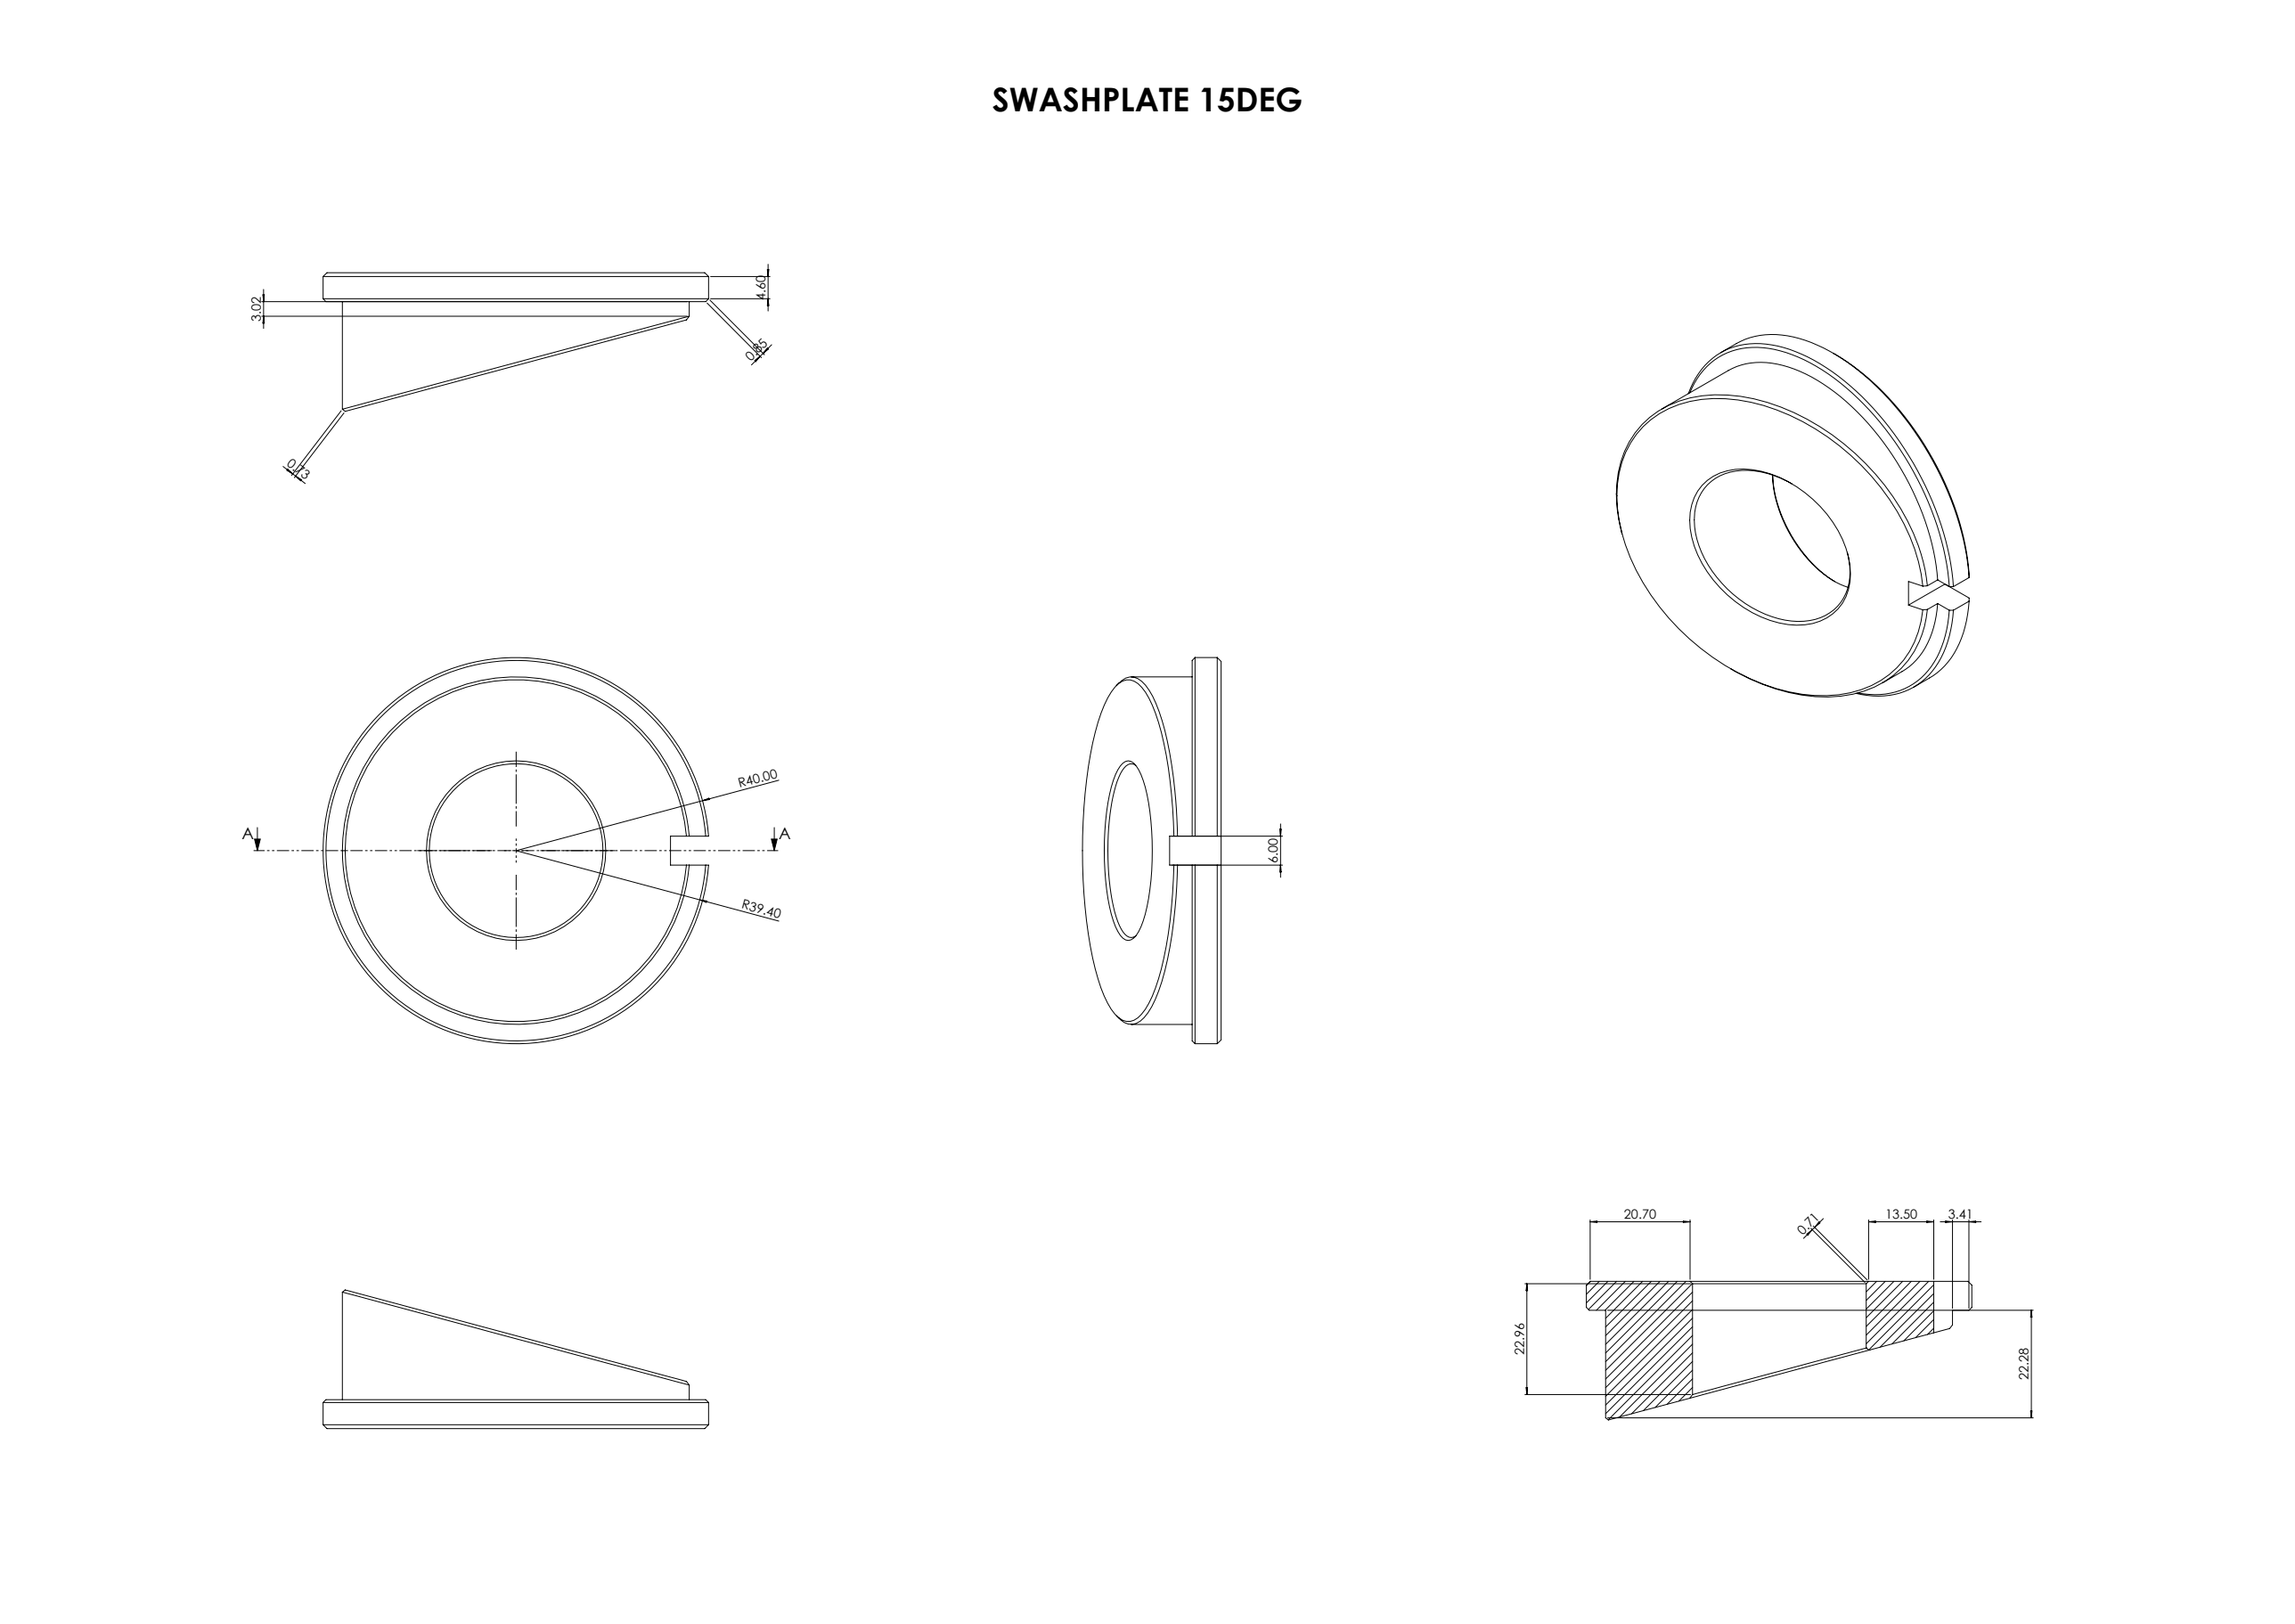
ISO-10303-21;
HEADER;
/* Generated by software containing ST-Developer
 * from STEP Tools, Inc. (www.steptools.com) 
 */

FILE_DESCRIPTION(
/* description */ (''),
/* implementation_level */ '2;1');

FILE_NAME(
/* name */ '10_Swashplate_15deg.step',
/* time_stamp */ '2026-10-23T00:52:27+05:00',
/* author */ (''),
/* organization */ (''),
/* preprocessor_version */ 'ST-DEVELOPER v20.2',
/* originating_system */ 'Autodesk Translation Framework v15.15.0.0',
/* authorisation */ '');

FILE_SCHEMA (('AUTOMOTIVE_DESIGN { 1 0 10303 214 3 1 1 }'));
ENDSEC;

DATA;
#10=MECHANICAL_DESIGN_GEOMETRIC_PRESENTATION_REPRESENTATION('',(#1550),#59204);
#314=B_SPLINE_SURFACE_WITH_KNOTS('',3,3,((#30941,#30942,#30943,#30944,#30945,
#30946,#30947,#30948,#30949,#30950),(#30951,#30952,#30953,#30954,#30955,
#30956,#30957,#30958,#30959,#30960),(#30961,#30962,#30963,#30964,#30965,
#30966,#30967,#30968,#30969,#30970),(#30971,#30972,#30973,#30974,#30975,
#30976,#30977,#30978,#30979,#30980)),.UNSPECIFIED.,.F.,.F.,.F.,(4,4),(4,
1,1,1,1,1,1,4),(0.,1.),(0.0830596749235681,0.519992957590172,0.956926240256775,
1.39385952292338,1.83079280558998,2.26772608825659,2.70465937092319,3.14159265358979),
 .UNSPECIFIED.);
#315=B_SPLINE_SURFACE_WITH_KNOTS('',3,3,((#31030,#31031,#31032,#31033,#31034,
#31035,#31036,#31037,#31038,#31039),(#31040,#31041,#31042,#31043,#31044,
#31045,#31046,#31047,#31048,#31049),(#31050,#31051,#31052,#31053,#31054,
#31055,#31056,#31057,#31058,#31059),(#31060,#31061,#31062,#31063,#31064,
#31065,#31066,#31067,#31068,#31069)),.UNSPECIFIED.,.F.,.F.,.F.,(4,4),(4,
1,1,1,1,1,1,4),(0.,1.),(-3.14159265358979,-2.70465937092292,-2.26772608825605,
-1.83079280558918,-1.39385952292231,-0.95692624025544,-0.519992957588569,
-0.083059674921698),.UNSPECIFIED.);
#316=B_SPLINE_SURFACE_WITH_KNOTS('',3,3,((#31111,#31112,#31113,#31114,#31115,
#31116,#31117,#31118,#31119,#31120,#31121,#31122,#31123,#31124,#31125,#31126,
#31127),(#31128,#31129,#31130,#31131,#31132,#31133,#31134,#31135,#31136,
#31137,#31138,#31139,#31140,#31141,#31142,#31143,#31144),(#31145,#31146,
#31147,#31148,#31149,#31150,#31151,#31152,#31153,#31154,#31155,#31156,#31157,
#31158,#31159,#31160,#31161),(#31162,#31163,#31164,#31165,#31166,#31167,
#31168,#31169,#31170,#31171,#31172,#31173,#31174,#31175,#31176,#31177,#31178)),
 .UNSPECIFIED.,.F.,.T.,.F.,(4,4),(4,1,1,1,1,1,1,1,1,1,1,1,1,1,4),(0.,1.),
(-3.14159265358979,-2.69279370307697,-2.24399475256414,-1.79519580205131,
-1.34639685153848,-1.0471975511966,-0.448798950512828,-0.149599650170943,
0.448798950512828,0.747998250854713,1.34639685153848,1.64559615188037,2.24399475256414,
2.69279370307697,3.14159265358979),.UNSPECIFIED.);
#569=B_SPLINE_CURVE_WITH_KNOTS('',3,(#30893,#30894,#30895,#30896,#30897,
#30898),.UNSPECIFIED.,.F.,.F.,(4,2,4),(-0.0953956468456381,-0.0476986988383283,
0.),.UNSPECIFIED.);
#570=B_SPLINE_CURVE_WITH_KNOTS('',3,(#30921,#30922,#30923,#30924,#30925,
#30926),.UNSPECIFIED.,.F.,.F.,(4,2,4),(-0.0953955489316151,-0.0476968906569989,
0.),.UNSPECIFIED.);
#571=B_SPLINE_CURVE_WITH_KNOTS('',3,(#30982,#30983,#30984,#30985,#30986,
#30987,#30988,#30989,#30990,#30991),.UNSPECIFIED.,.F.,.F.,(4,1,1,1,1,1,
1,4),(0.0848980286013396,0.519992957590172,0.956926240256775,1.39385952292338,
1.83079280558998,2.26772608825659,2.70465937092319,3.14159265358979),
 .UNSPECIFIED.);
#572=B_SPLINE_CURVE_WITH_KNOTS('',3,(#30994,#30995,#30996,#30997,#30998,
#30999,#31000,#31001,#31002,#31003),.UNSPECIFIED.,.F.,.F.,(4,1,1,1,1,1,
1,4),(-3.14159265358979,-2.70465937092319,-2.26772608825659,-1.83079280558998,
-1.39385952292338,-0.956926240256775,-0.519992957590172,-0.0830596749235681),
 .UNSPECIFIED.);
#573=B_SPLINE_CURVE_WITH_KNOTS('',3,(#31012,#31013,#31014,#31015,#31016,
#31017,#31018,#31019,#31020,#31021,#31022,#31023,#31024,#31025,#31026,#31027,
#31028),.UNSPECIFIED.,.T.,.F.,(4,1,1,1,1,1,1,1,1,1,1,1,1,1,4),(-3.14159265358979,
-2.69279370307697,-2.24399475256414,-1.64559615188037,-1.34639685153848,
-0.747998250854713,-0.448798950512828,0.149599650170943,0.448798950512828,
1.0471975511966,1.34639685153848,1.79519580205131,2.24399475256414,2.69279370307697,
3.14159265358979),.UNSPECIFIED.);
#574=B_SPLINE_CURVE_WITH_KNOTS('',3,(#31070,#31071,#31072,#31073,#31074,
#31075,#31076,#31077,#31078,#31079),.UNSPECIFIED.,.F.,.F.,(4,1,1,1,1,1,
1,4),(0.083059674921698,0.519992957588569,0.95692624025544,1.39385952292231,
1.83079280558918,2.26772608825605,2.70465937092292,3.14159265358979),
 .UNSPECIFIED.);
#575=B_SPLINE_CURVE_WITH_KNOTS('',3,(#31080,#31081,#31082,#31083,#31084,
#31085,#31086,#31087,#31088,#31089),.UNSPECIFIED.,.F.,.F.,(4,1,1,1,1,1,
1,4),(-3.14159265358979,-2.70465937092292,-2.26772608825605,-1.83079280558918,
-1.39385952292231,-0.95692624025544,-0.519992957588569,-0.0848980305822978),
 .UNSPECIFIED.);
#576=B_SPLINE_CURVE_WITH_KNOTS('',3,(#31092,#31093,#31094,#31095,#31096,
#31097,#31098,#31099,#31100,#31101,#31102,#31103,#31104,#31105,#31106,#31107,
#31108),.UNSPECIFIED.,.T.,.F.,(4,1,1,1,1,1,1,1,1,1,1,1,1,1,4),(-3.14159265358979,
-2.69279370307697,-2.24399475256414,-1.79519580205131,-1.34639685153848,
-1.0471975511966,-0.448798950512828,-0.149599650170943,0.448798950512828,
0.747998250854713,1.34639685153848,1.64559615188037,2.24399475256414,2.69279370307697,
3.14159265358979),.UNSPECIFIED.);
#1452=(
BOUNDED_CURVE()
B_SPLINE_CURVE(2,(#30883,#30884,#30885),.UNSPECIFIED.,.F.,.F.)
B_SPLINE_CURVE_WITH_KNOTS((3,3),(0.,0.113300250597084),.UNSPECIFIED.)
CURVE()
GEOMETRIC_REPRESENTATION_ITEM()
RATIONAL_B_SPLINE_CURVE((1.,1.00005131202982,1.))
REPRESENTATION_ITEM('')
);
#1453=(
BOUNDED_CURVE()
B_SPLINE_CURVE(2,(#30909,#30910,#30911),.UNSPECIFIED.,.F.,.F.)
B_SPLINE_CURVE_WITH_KNOTS((3,3),(0.,0.113300250597084),.UNSPECIFIED.)
CURVE()
GEOMETRIC_REPRESENTATION_ITEM()
RATIONAL_B_SPLINE_CURVE((1.,1.00005131202982,1.))
REPRESENTATION_ITEM('')
);
#1510=SHAPE_REPRESENTATION_RELATIONSHIP('SRR','None',#59299,#1530);
#1530=ADVANCED_BREP_SHAPE_REPRESENTATION('',(#1577),#59186);
#1550=STYLED_ITEM('',(#59572),#1577);
#1577=MANIFOLD_SOLID_BREP('Swashplate',#22806);
#1622=FACE_BOUND('',#4044,.T.);
#1623=FACE_BOUND('',#4051,.T.);
#1815=PLANE('',#23146);
#1816=PLANE('',#23147);
#1817=PLANE('',#23148);
#1818=PLANE('',#23149);
#1819=PLANE('',#23158);
#1820=PLANE('',#23165);
#2422=CYLINDRICAL_SURFACE('',#23157,1.8);
#2423=CYLINDRICAL_SURFACE('',#23159,3.6);
#2424=CYLINDRICAL_SURFACE('',#23161,4.);
#2712=FACE_OUTER_BOUND('',#4040,.T.);
#2713=FACE_OUTER_BOUND('',#4041,.T.);
#2714=FACE_OUTER_BOUND('',#4042,.T.);
#2715=FACE_OUTER_BOUND('',#4043,.T.);
#2716=FACE_OUTER_BOUND('',#4045,.T.);
#2717=FACE_OUTER_BOUND('',#4046,.T.);
#2718=FACE_OUTER_BOUND('',#4047,.T.);
#2719=FACE_OUTER_BOUND('',#4048,.T.);
#2720=FACE_OUTER_BOUND('',#4049,.T.);
#2721=FACE_OUTER_BOUND('',#4050,.T.);
#2722=FACE_OUTER_BOUND('',#4052,.T.);
#2723=FACE_OUTER_BOUND('',#4053,.T.);
#2724=FACE_OUTER_BOUND('',#4054,.T.);
#2725=FACE_OUTER_BOUND('',#4055,.T.);
#2726=FACE_OUTER_BOUND('',#4056,.T.);
#4040=EDGE_LOOP('',(#14842,#14843,#14844,#14845,#14846,#14847,#14848,#14849,
#14850));
#4041=EDGE_LOOP('',(#14851,#14852,#14853,#14854,#14855,#14856,#14857,#14858,
#14859));
#4042=EDGE_LOOP('',(#14860,#14861,#14862,#14863));
#4043=EDGE_LOOP('',(#14864,#14865,#14866,#14867));
#4044=EDGE_LOOP('',(#14868));
#4045=EDGE_LOOP('',(#14869,#14870,#14871,#14872));
#4046=EDGE_LOOP('',(#14873,#14874,#14875,#14876));
#4047=EDGE_LOOP('',(#14877,#14878,#14879,#14880,#14881));
#4048=EDGE_LOOP('',(#14882,#14883,#14884,#14885,#14886));
#4049=EDGE_LOOP('',(#14887,#14888,#14889,#14890));
#4050=EDGE_LOOP('',(#14891,#14892,#14893,#14894,#14895));
#4051=EDGE_LOOP('',(#14896));
#4052=EDGE_LOOP('',(#14897,#14898,#14899,#14900,#14901));
#4053=EDGE_LOOP('',(#14902,#14903,#14904,#14905));
#4054=EDGE_LOOP('',(#14906,#14907,#14908,#14909));
#4055=EDGE_LOOP('',(#14910,#14911,#14912,#14913));
#4056=EDGE_LOOP('',(#14914,#14915,#14916,#14917));
#5526=LINE('',#30887,#6959);
#5527=LINE('',#30889,#6960);
#5528=LINE('',#30891,#6961);
#5529=LINE('',#30900,#6962);
#5530=LINE('',#30902,#6963);
#5531=LINE('',#30904,#6964);
#5532=LINE('',#30905,#6965);
#5533=LINE('',#30913,#6966);
#5534=LINE('',#30915,#6967);
#5535=LINE('',#30917,#6968);
#5536=LINE('',#30919,#6969);
#5537=LINE('',#30928,#6970);
#5538=LINE('',#30930,#6971);
#5539=LINE('',#30931,#6972);
#5540=LINE('',#30933,#6973);
#5541=LINE('',#30934,#6974);
#5542=LINE('',#30993,#6975);
#5543=LINE('',#31006,#6976);
#5544=LINE('',#31029,#6977);
#5545=LINE('',#31179,#6978);
#6959=VECTOR('',#25356,1.);
#6960=VECTOR('',#25357,1.);
#6961=VECTOR('',#25358,1.);
#6962=VECTOR('',#25359,1.);
#6963=VECTOR('',#25360,1.);
#6964=VECTOR('',#25361,1.);
#6965=VECTOR('',#25362,1.);
#6966=VECTOR('',#25365,1.);
#6967=VECTOR('',#25366,1.);
#6968=VECTOR('',#25367,1.);
#6969=VECTOR('',#25368,1.);
#6970=VECTOR('',#25369,1.);
#6971=VECTOR('',#25370,1.);
#6972=VECTOR('',#25371,1.);
#6973=VECTOR('',#25374,1.);
#6974=VECTOR('',#25375,1.);
#6975=VECTOR('',#25386,1.);
#6976=VECTOR('',#25389,1.825);
#6977=VECTOR('',#25396,1.8);
#6978=VECTOR('',#25403,1.);
#8410=CIRCLE('',#23150,3.92);
#8411=CIRCLE('',#23151,1.85);
#8412=CIRCLE('',#23153,4.);
#8413=CIRCLE('',#23155,1.8);
#8414=CIRCLE('',#23156,1.8);
#8415=CIRCLE('',#23160,3.6);
#8416=CIRCLE('',#23162,4.);
#8417=CIRCLE('',#23164,3.94);
#9244=VERTEX_POINT('',#30881);
#9245=VERTEX_POINT('',#30882);
#9246=VERTEX_POINT('',#30886);
#9247=VERTEX_POINT('',#30888);
#9248=VERTEX_POINT('',#30890);
#9249=VERTEX_POINT('',#30892);
#9250=VERTEX_POINT('',#30899);
#9251=VERTEX_POINT('',#30901);
#9252=VERTEX_POINT('',#30903);
#9253=VERTEX_POINT('',#30907);
#9254=VERTEX_POINT('',#30908);
#9255=VERTEX_POINT('',#30912);
#9256=VERTEX_POINT('',#30914);
#9257=VERTEX_POINT('',#30916);
#9258=VERTEX_POINT('',#30918);
#9259=VERTEX_POINT('',#30920);
#9260=VERTEX_POINT('',#30927);
#9261=VERTEX_POINT('',#30929);
#9262=VERTEX_POINT('',#30937);
#9263=VERTEX_POINT('',#30981);
#9264=VERTEX_POINT('',#30992);
#9265=VERTEX_POINT('',#31005);
#9266=VERTEX_POINT('',#31007);
#9267=VERTEX_POINT('',#31011);
#9268=VERTEX_POINT('',#31091);
#11425=EDGE_CURVE('',#9244,#9245,#1452,.T.);
#11426=EDGE_CURVE('',#9246,#9244,#5526,.T.);
#11427=EDGE_CURVE('',#9246,#9247,#5527,.T.);
#11428=EDGE_CURVE('',#9248,#9247,#5528,.T.);
#11429=EDGE_CURVE('',#9249,#9248,#569,.T.);
#11430=EDGE_CURVE('',#9250,#9249,#5529,.T.);
#11431=EDGE_CURVE('',#9251,#9250,#5530,.T.);
#11432=EDGE_CURVE('',#9252,#9251,#5531,.T.);
#11433=EDGE_CURVE('',#9245,#9252,#5532,.T.);
#11434=EDGE_CURVE('',#9253,#9254,#1453,.T.);
#11435=EDGE_CURVE('',#9255,#9253,#5533,.T.);
#11436=EDGE_CURVE('',#9256,#9255,#5534,.T.);
#11437=EDGE_CURVE('',#9257,#9256,#5535,.T.);
#11438=EDGE_CURVE('',#9258,#9257,#5536,.T.);
#11439=EDGE_CURVE('',#9259,#9258,#570,.T.);
#11440=EDGE_CURVE('',#9260,#9259,#5537,.T.);
#11441=EDGE_CURVE('',#9261,#9260,#5538,.T.);
#11442=EDGE_CURVE('',#9254,#9261,#5539,.T.);
#11443=EDGE_CURVE('',#9247,#9260,#5540,.T.);
#11444=EDGE_CURVE('',#9261,#9246,#5541,.T.);
#11445=EDGE_CURVE('',#9254,#9244,#8410,.T.);
#11446=EDGE_CURVE('',#9262,#9262,#8411,.T.);
#11447=EDGE_CURVE('',#9253,#9245,#8412,.T.);
#11448=EDGE_CURVE('',#9248,#9263,#571,.T.);
#11449=EDGE_CURVE('',#9264,#9263,#5542,.T.);
#11450=EDGE_CURVE('',#9264,#9249,#572,.T.);
#11451=EDGE_CURVE('',#9262,#9265,#5543,.T.);
#11452=EDGE_CURVE('',#9265,#9266,#8413,.T.);
#11453=EDGE_CURVE('',#9266,#9265,#8414,.T.);
#11454=EDGE_CURVE('',#9267,#9267,#573,.T.);
#11455=EDGE_CURVE('',#9267,#9266,#5544,.T.);
#11456=EDGE_CURVE('',#9258,#9264,#574,.T.);
#11457=EDGE_CURVE('',#9263,#9259,#575,.T.);
#11458=EDGE_CURVE('',#9268,#9268,#576,.T.);
#11459=EDGE_CURVE('',#9257,#9250,#8415,.T.);
#11460=EDGE_CURVE('',#9267,#9268,#5545,.T.);
#11461=EDGE_CURVE('',#9255,#9252,#8416,.T.);
#11462=EDGE_CURVE('',#9256,#9251,#8417,.T.);
#14842=ORIENTED_EDGE('',*,*,#11425,.F.);
#14843=ORIENTED_EDGE('',*,*,#11426,.F.);
#14844=ORIENTED_EDGE('',*,*,#11427,.T.);
#14845=ORIENTED_EDGE('',*,*,#11428,.F.);
#14846=ORIENTED_EDGE('',*,*,#11429,.F.);
#14847=ORIENTED_EDGE('',*,*,#11430,.F.);
#14848=ORIENTED_EDGE('',*,*,#11431,.F.);
#14849=ORIENTED_EDGE('',*,*,#11432,.F.);
#14850=ORIENTED_EDGE('',*,*,#11433,.F.);
#14851=ORIENTED_EDGE('',*,*,#11434,.F.);
#14852=ORIENTED_EDGE('',*,*,#11435,.F.);
#14853=ORIENTED_EDGE('',*,*,#11436,.F.);
#14854=ORIENTED_EDGE('',*,*,#11437,.F.);
#14855=ORIENTED_EDGE('',*,*,#11438,.F.);
#14856=ORIENTED_EDGE('',*,*,#11439,.F.);
#14857=ORIENTED_EDGE('',*,*,#11440,.F.);
#14858=ORIENTED_EDGE('',*,*,#11441,.F.);
#14859=ORIENTED_EDGE('',*,*,#11442,.F.);
#14860=ORIENTED_EDGE('',*,*,#11443,.F.);
#14861=ORIENTED_EDGE('',*,*,#11427,.F.);
#14862=ORIENTED_EDGE('',*,*,#11444,.F.);
#14863=ORIENTED_EDGE('',*,*,#11441,.T.);
#14864=ORIENTED_EDGE('',*,*,#11442,.T.);
#14865=ORIENTED_EDGE('',*,*,#11444,.T.);
#14866=ORIENTED_EDGE('',*,*,#11426,.T.);
#14867=ORIENTED_EDGE('',*,*,#11445,.F.);
#14868=ORIENTED_EDGE('',*,*,#11446,.F.);
#14869=ORIENTED_EDGE('',*,*,#11434,.T.);
#14870=ORIENTED_EDGE('',*,*,#11445,.T.);
#14871=ORIENTED_EDGE('',*,*,#11425,.T.);
#14872=ORIENTED_EDGE('',*,*,#11447,.F.);
#14873=ORIENTED_EDGE('',*,*,#11429,.T.);
#14874=ORIENTED_EDGE('',*,*,#11448,.T.);
#14875=ORIENTED_EDGE('',*,*,#11449,.F.);
#14876=ORIENTED_EDGE('',*,*,#11450,.T.);
#14877=ORIENTED_EDGE('',*,*,#11446,.T.);
#14878=ORIENTED_EDGE('',*,*,#11451,.T.);
#14879=ORIENTED_EDGE('',*,*,#11452,.T.);
#14880=ORIENTED_EDGE('',*,*,#11453,.T.);
#14881=ORIENTED_EDGE('',*,*,#11451,.F.);
#14882=ORIENTED_EDGE('',*,*,#11454,.F.);
#14883=ORIENTED_EDGE('',*,*,#11455,.T.);
#14884=ORIENTED_EDGE('',*,*,#11452,.F.);
#14885=ORIENTED_EDGE('',*,*,#11453,.F.);
#14886=ORIENTED_EDGE('',*,*,#11455,.F.);
#14887=ORIENTED_EDGE('',*,*,#11439,.T.);
#14888=ORIENTED_EDGE('',*,*,#11456,.T.);
#14889=ORIENTED_EDGE('',*,*,#11449,.T.);
#14890=ORIENTED_EDGE('',*,*,#11457,.T.);
#14891=ORIENTED_EDGE('',*,*,#11440,.T.);
#14892=ORIENTED_EDGE('',*,*,#11457,.F.);
#14893=ORIENTED_EDGE('',*,*,#11448,.F.);
#14894=ORIENTED_EDGE('',*,*,#11428,.T.);
#14895=ORIENTED_EDGE('',*,*,#11443,.T.);
#14896=ORIENTED_EDGE('',*,*,#11458,.F.);
#14897=ORIENTED_EDGE('',*,*,#11438,.T.);
#14898=ORIENTED_EDGE('',*,*,#11459,.T.);
#14899=ORIENTED_EDGE('',*,*,#11430,.T.);
#14900=ORIENTED_EDGE('',*,*,#11450,.F.);
#14901=ORIENTED_EDGE('',*,*,#11456,.F.);
#14902=ORIENTED_EDGE('',*,*,#11460,.T.);
#14903=ORIENTED_EDGE('',*,*,#11458,.T.);
#14904=ORIENTED_EDGE('',*,*,#11460,.F.);
#14905=ORIENTED_EDGE('',*,*,#11454,.T.);
#14906=ORIENTED_EDGE('',*,*,#11435,.T.);
#14907=ORIENTED_EDGE('',*,*,#11447,.T.);
#14908=ORIENTED_EDGE('',*,*,#11433,.T.);
#14909=ORIENTED_EDGE('',*,*,#11461,.F.);
#14910=ORIENTED_EDGE('',*,*,#11436,.T.);
#14911=ORIENTED_EDGE('',*,*,#11461,.T.);
#14912=ORIENTED_EDGE('',*,*,#11432,.T.);
#14913=ORIENTED_EDGE('',*,*,#11462,.F.);
#14914=ORIENTED_EDGE('',*,*,#11437,.T.);
#14915=ORIENTED_EDGE('',*,*,#11462,.T.);
#14916=ORIENTED_EDGE('',*,*,#11431,.T.);
#14917=ORIENTED_EDGE('',*,*,#11459,.F.);
#21339=CONICAL_SURFACE('',#23152,3.96,0.785398163397457);
#21340=CONICAL_SURFACE('',#23154,1.825,0.785398163397442);
#21341=CONICAL_SURFACE('',#23163,3.97,0.785398163397445);
#21542=ADVANCED_FACE('',(#2712),#1815,.F.);
#21543=ADVANCED_FACE('',(#2713),#1816,.F.);
#21544=ADVANCED_FACE('',(#2714),#1817,.F.);
#21545=ADVANCED_FACE('',(#2715,#1622),#1818,.T.);
#21546=ADVANCED_FACE('',(#2716),#21339,.T.);
#21547=ADVANCED_FACE('',(#2717),#314,.T.);
#21548=ADVANCED_FACE('',(#2718),#21340,.F.);
#21549=ADVANCED_FACE('',(#2719),#2422,.F.);
#21550=ADVANCED_FACE('',(#2720),#315,.T.);
#21551=ADVANCED_FACE('',(#2721,#1623),#1819,.F.);
#21552=ADVANCED_FACE('',(#2722),#2423,.T.);
#21553=ADVANCED_FACE('',(#2723),#316,.T.);
#21554=ADVANCED_FACE('',(#2724),#2424,.T.);
#21555=ADVANCED_FACE('',(#2725),#21341,.T.);
#21556=ADVANCED_FACE('',(#2726),#1820,.T.);
#22806=CLOSED_SHELL('',(#21542,#21543,#21544,#21545,#21546,#21547,#21548,
#21549,#21550,#21551,#21552,#21553,#21554,#21555,#21556));
#23145=AXIS2_PLACEMENT_3D('',#30879,#25352,#25353);
#23146=AXIS2_PLACEMENT_3D('',#30880,#25354,#25355);
#23147=AXIS2_PLACEMENT_3D('',#30906,#25363,#25364);
#23148=AXIS2_PLACEMENT_3D('',#30932,#25372,#25373);
#23149=AXIS2_PLACEMENT_3D('',#30935,#25376,#25377);
#23150=AXIS2_PLACEMENT_3D('',#30936,#25378,#25379);
#23151=AXIS2_PLACEMENT_3D('',#30938,#25380,#25381);
#23152=AXIS2_PLACEMENT_3D('',#30939,#25382,#25383);
#23153=AXIS2_PLACEMENT_3D('',#30940,#25384,#25385);
#23154=AXIS2_PLACEMENT_3D('',#31004,#25387,#25388);
#23155=AXIS2_PLACEMENT_3D('',#31008,#25390,#25391);
#23156=AXIS2_PLACEMENT_3D('',#31009,#25392,#25393);
#23157=AXIS2_PLACEMENT_3D('',#31010,#25394,#25395);
#23158=AXIS2_PLACEMENT_3D('',#31090,#25397,#25398);
#23159=AXIS2_PLACEMENT_3D('',#31109,#25399,#25400);
#23160=AXIS2_PLACEMENT_3D('',#31110,#25401,#25402);
#23161=AXIS2_PLACEMENT_3D('',#31180,#25404,#25405);
#23162=AXIS2_PLACEMENT_3D('',#31181,#25406,#25407);
#23163=AXIS2_PLACEMENT_3D('',#31182,#25408,#25409);
#23164=AXIS2_PLACEMENT_3D('',#31183,#25410,#25411);
#23165=AXIS2_PLACEMENT_3D('',#31184,#25412,#25413);
#25352=DIRECTION('axis',(0.,0.,1.));
#25353=DIRECTION('refdir',(1.,0.,0.));
#25354=DIRECTION('center_axis',(0.,-1.,0.));
#25355=DIRECTION('ref_axis',(1.,0.,0.));
#25356=DIRECTION('',(1.,0.,0.));
#25357=DIRECTION('',(0.,0.,1.));
#25358=DIRECTION('',(-0.965925826289068,0.,0.258819045102521));
#25359=DIRECTION('',(0.,0.,1.));
#25360=DIRECTION('',(-1.,0.,0.));
#25361=DIRECTION('',(-0.708118460127311,0.,0.706093652730943));
#25362=DIRECTION('',(0.,0.,1.));
#25363=DIRECTION('center_axis',(0.,1.,0.));
#25364=DIRECTION('ref_axis',(-1.,0.,0.));
#25365=DIRECTION('',(0.,0.,-1.));
#25366=DIRECTION('',(0.708118460127311,0.,-0.706093652730943));
#25367=DIRECTION('',(1.,0.,0.));
#25368=DIRECTION('',(0.,0.,-1.));
#25369=DIRECTION('',(0.965925826289068,0.,-0.258819045102521));
#25370=DIRECTION('',(0.,0.,1.));
#25371=DIRECTION('',(-1.,0.,0.));
#25372=DIRECTION('center_axis',(-1.,0.,0.));
#25373=DIRECTION('ref_axis',(0.,-1.,0.));
#25374=DIRECTION('',(0.,1.,0.));
#25375=DIRECTION('',(0.,-1.,0.));
#25376=DIRECTION('center_axis',(0.,0.,-1.));
#25377=DIRECTION('ref_axis',(-1.,0.,0.));
#25378=DIRECTION('center_axis',(0.,0.,1.));
#25379=DIRECTION('ref_axis',(1.,0.,0.));
#25380=DIRECTION('center_axis',(0.,0.,-1.));
#25381=DIRECTION('ref_axis',(-1.,0.,0.));
#25382=DIRECTION('center_axis',(0.,0.,1.));
#25383=DIRECTION('ref_axis',(-1.,1.22464679914735E-16,0.));
#25384=DIRECTION('center_axis',(0.,0.,1.));
#25385=DIRECTION('ref_axis',(1.,0.,0.));
#25386=DIRECTION('',(0.793353340291233,-9.91880824887135E-15,0.608761429008723));
#25387=DIRECTION('center_axis',(0.,0.,-1.));
#25388=DIRECTION('ref_axis',(-1.,0.,0.));
#25389=DIRECTION('',(-0.707106781186543,8.65956056235487E-17,0.707106781186552));
#25390=DIRECTION('center_axis',(0.,0.,1.));
#25391=DIRECTION('ref_axis',(-1.,0.,0.));
#25392=DIRECTION('center_axis',(0.,0.,1.));
#25393=DIRECTION('ref_axis',(-1.,0.,0.));
#25394=DIRECTION('center_axis',(0.,0.,1.));
#25395=DIRECTION('ref_axis',(1.,0.,0.));
#25396=DIRECTION('',(0.,0.,-1.));
#25397=DIRECTION('center_axis',(-0.258819045102521,0.,-0.965925826289068));
#25398=DIRECTION('ref_axis',(-0.965925826289068,0.,0.258819045102521));
#25399=DIRECTION('center_axis',(0.,0.,1.));
#25400=DIRECTION('ref_axis',(-1.,9.39371143512797E-13,0.));
#25401=DIRECTION('center_axis',(0.,0.,1.));
#25402=DIRECTION('ref_axis',(1.,0.,0.));
#25403=DIRECTION('',(-0.608761429008725,-7.99043500659679E-17,0.793353340291232));
#25404=DIRECTION('center_axis',(0.,0.,1.));
#25405=DIRECTION('ref_axis',(-1.,1.22464679914735E-16,0.));
#25406=DIRECTION('center_axis',(0.,0.,1.));
#25407=DIRECTION('ref_axis',(1.,0.,0.));
#25408=DIRECTION('center_axis',(0.,0.,-1.));
#25409=DIRECTION('ref_axis',(-1.,1.22464679914735E-16,0.));
#25410=DIRECTION('center_axis',(0.,0.,1.));
#25411=DIRECTION('ref_axis',(1.,0.,0.));
#25412=DIRECTION('center_axis',(0.,0.,1.));
#25413=DIRECTION('ref_axis',(1.,0.,0.));
#30879=CARTESIAN_POINT('',(0.,0.,0.));
#30880=CARTESIAN_POINT('Origin',(3.2,-0.3,-9.2));
#30881=CARTESIAN_POINT('',(3.90850354995361,-0.3,-9.2));
#30882=CARTESIAN_POINT('',(3.98873413503583,-0.3,-9.12));
#30883=CARTESIAN_POINT('Ctrl Pts',(3.90850354995361,-0.3,-9.2));
#30884=CARTESIAN_POINT('Ctrl Pts',(3.94821363792151,-0.3,-9.16040637250214));
#30885=CARTESIAN_POINT('Ctrl Pts',(3.98873413503583,-0.3,-9.12));
#30886=CARTESIAN_POINT('',(3.2,-0.3,-9.2));
#30887=CARTESIAN_POINT('',(3.56,-0.3,-9.2));
#30888=CARTESIAN_POINT('',(3.2,-0.3,-8.13377950492769));
#30889=CARTESIAN_POINT('',(3.2,-0.3,-9.2));
#30890=CARTESIAN_POINT('',(3.52930206283097,-0.299999999999879,-8.22201572672916));
#30891=CARTESIAN_POINT('',(4.23327756188404,-0.3,-8.41064539319172));
#30892=CARTESIAN_POINT('',(3.58747822293044,-0.299999999999851,-8.29761887140429));
#30893=CARTESIAN_POINT('Ctrl Pts',(3.58747822293042,-0.299999999999999,
-8.29761887140429));
#30894=CARTESIAN_POINT('Ctrl Pts',(3.57778261485426,-0.299999999999999,
-8.28501838269504));
#30895=CARTESIAN_POINT('Ctrl Pts',(3.56808690015176,-0.300000000000001,
-8.2724180070262));
#30896=CARTESIAN_POINT('Ctrl Pts',(3.54869482834287,-0.300000000000001,
-8.2472169321301));
#30897=CARTESIAN_POINT('Ctrl Pts',(3.53899853098755,-0.300000000000002,
-8.23461631057127));
#30898=CARTESIAN_POINT('Ctrl Pts',(3.52930206283095,-0.300000000000002,
-8.22201572672915));
#30899=CARTESIAN_POINT('',(3.58747822293042,-0.3,-8.6));
#30900=CARTESIAN_POINT('',(3.58747822293042,-0.3,-6.8));
#30901=CARTESIAN_POINT('',(3.92856207791095,-0.3,-8.6));
#30902=CARTESIAN_POINT('',(3.4,-0.3,-8.6));
#30903=CARTESIAN_POINT('',(3.98873413503583,-0.3,-8.66));
#30904=CARTESIAN_POINT('',(3.95864810647339,-0.3,-8.63));
#30905=CARTESIAN_POINT('',(3.98873413503583,-0.3,-8.89));
#30906=CARTESIAN_POINT('Origin',(4.1,0.3,-9.2));
#30907=CARTESIAN_POINT('',(3.98873413503583,0.3,-9.12));
#30908=CARTESIAN_POINT('',(3.90850354995361,0.3,-9.2));
#30909=CARTESIAN_POINT('Ctrl Pts',(3.98873413503583,0.3,-9.12));
#30910=CARTESIAN_POINT('Ctrl Pts',(3.94821363792151,0.3,-9.16040637250214));
#30911=CARTESIAN_POINT('Ctrl Pts',(3.90850354995361,0.3,-9.2));
#30912=CARTESIAN_POINT('',(3.98873413503583,0.3,-8.66));
#30913=CARTESIAN_POINT('',(3.98873413503583,0.3,-8.89));
#30914=CARTESIAN_POINT('',(3.92856207791095,0.3,-8.6));
#30915=CARTESIAN_POINT('',(3.95864810647339,0.3,-8.63));
#30916=CARTESIAN_POINT('',(3.58747822293042,0.3,-8.6));
#30917=CARTESIAN_POINT('',(3.85,0.3,-8.6));
#30918=CARTESIAN_POINT('',(3.58747822293156,0.299999999993159,-8.29761887140459));
#30919=CARTESIAN_POINT('',(3.58747822293042,0.3,-6.8));
#30920=CARTESIAN_POINT('',(3.52930206283204,0.299999999993599,-8.22201572672944));
#30921=CARTESIAN_POINT('Ctrl Pts',(3.52930206283095,0.300000000000001,-8.22201572672915));
#30922=CARTESIAN_POINT('Ctrl Pts',(3.53899853259429,0.300000000000001,-8.23461631265923));
#30923=CARTESIAN_POINT('Ctrl Pts',(3.54869483155032,0.300000000000001,-8.24721693629827));
#30924=CARTESIAN_POINT('Ctrl Pts',(3.56808690349722,0.300000000000001,-8.2724180113739));
#30925=CARTESIAN_POINT('Ctrl Pts',(3.57778261657339,0.299999999999999,-8.28501838492923));
#30926=CARTESIAN_POINT('Ctrl Pts',(3.58747822293042,0.299999999999999,-8.29761887140429));
#30927=CARTESIAN_POINT('',(3.2,0.3,-8.13377950492769));
#30928=CARTESIAN_POINT('',(4.65313327773554,0.3,-8.52314539319172));
#30929=CARTESIAN_POINT('',(3.2,0.3,-9.2));
#30930=CARTESIAN_POINT('',(3.2,0.3,-9.2));
#30931=CARTESIAN_POINT('',(4.01,0.3,-9.2));
#30932=CARTESIAN_POINT('Origin',(3.2,0.3,-9.2));
#30933=CARTESIAN_POINT('',(3.2,0.15,-8.13377950492769));
#30934=CARTESIAN_POINT('',(3.2,0.15,-9.2));
#30935=CARTESIAN_POINT('Origin',(3.92,0.,-9.2));
#30936=CARTESIAN_POINT('Origin',(0.,0.,-9.2));
#30937=CARTESIAN_POINT('',(1.85,-2.2655965784226E-16,-9.2));
#30938=CARTESIAN_POINT('Origin',(0.,0.,-9.2));
#30939=CARTESIAN_POINT('Origin',(0.,0.,-9.16));
#30940=CARTESIAN_POINT('Origin',(0.,0.,-9.12));
#30941=CARTESIAN_POINT('Ctrl Pts',(3.58747822293043,-0.299999999999847,
-8.29761887140429));
#30942=CARTESIAN_POINT('Ctrl Pts',(3.54359058486425,-0.824819819394348,
-8.28591130419311));
#30943=CARTESIAN_POINT('Ctrl Pts',(3.22201167914007,-1.85462953693043,-8.20013753826912));
#30944=CARTESIAN_POINT('Ctrl Pts',(2.12984786621321,-3.04615572678008,-7.90851029361343));
#30945=CARTESIAN_POINT('Ctrl Pts',(0.638165371196739,-3.66186103320656,
-7.50952634922024));
#30946=CARTESIAN_POINT('Ctrl Pts',(-0.970794977809144,-3.58699051730416,
-7.0783176016057));
#30947=CARTESIAN_POINT('Ctrl Pts',(-2.39520557608279,-2.84138111621991,
-6.69582652891509));
#30948=CARTESIAN_POINT('Ctrl Pts',(-3.36945925169178,-1.56555438904003,
-6.43378922985514));
#30949=CARTESIAN_POINT('Ctrl Pts',(-3.6,-0.521978420795187,-6.37172499639606));
#30950=CARTESIAN_POINT('Ctrl Pts',(-3.6,1.15784830776718E-15,-6.37172499639606));
#30951=CARTESIAN_POINT('Ctrl Pts',(3.56826802079061,-0.297839652204228,
-8.27246655006857));
#30952=CARTESIAN_POINT('Ctrl Pts',(3.52475967172772,-0.81888729728801,-8.2608432497174));
#30953=CARTESIAN_POINT('Ctrl Pts',(3.20600009782036,-1.84143224327734,-8.17569390742104));
#30954=CARTESIAN_POINT('Ctrl Pts',(2.12230631674708,-3.02629090956407,-7.88599714528684));
#30955=CARTESIAN_POINT('Ctrl Pts',(0.640141493156845,-3.64055636684028,
-7.48932639476278));
#30956=CARTESIAN_POINT('Ctrl Pts',(-0.960725860124494,-3.56849488474166,
-7.06031586596521));
#30957=CARTESIAN_POINT('Ctrl Pts',(-2.37955235373569,-2.82823993196693,
-6.67959485067365));
#30958=CARTESIAN_POINT('Ctrl Pts',(-3.35076472884238,-1.55884475475421,
-6.41870140344638));
#30959=CARTESIAN_POINT('Ctrl Pts',(-3.58068148347422,-0.519743282796945,
-6.35690137729811));
#30960=CARTESIAN_POINT('Ctrl Pts',(-3.58068148347422,1.15118890346963E-15,
-6.35690137729811));
#30961=CARTESIAN_POINT('Ctrl Pts',(3.54905781865079,-0.295679304408609,
-8.24731422873286));
#30962=CARTESIAN_POINT('Ctrl Pts',(3.50592875859118,-0.812954775181674,
-8.23577519524169));
#30963=CARTESIAN_POINT('Ctrl Pts',(3.18998851650066,-1.82823494962424,-8.15125027657294));
#30964=CARTESIAN_POINT('Ctrl Pts',(2.11476476728094,-3.00642609234806,-7.86348399696027));
#30965=CARTESIAN_POINT('Ctrl Pts',(0.642117615116952,-3.61925170047399,
-7.46912644030531));
#30966=CARTESIAN_POINT('Ctrl Pts',(-0.950656742439843,-3.54999925217916,
-7.04231413032472));
#30967=CARTESIAN_POINT('Ctrl Pts',(-2.36389913138858,-2.81509874771395,
-6.6633631724322));
#30968=CARTESIAN_POINT('Ctrl Pts',(-3.33207020599299,-1.5521351204684,-6.40361357703761));
#30969=CARTESIAN_POINT('Ctrl Pts',(-3.56136296694844,-0.517508144798703,
-6.34207775820016));
#30970=CARTESIAN_POINT('Ctrl Pts',(-3.56136296694844,1.14452949917207E-15,
-6.34207775820016));
#30971=CARTESIAN_POINT('Ctrl Pts',(3.52984761651097,-0.29351895661299,-8.22216190739714));
#30972=CARTESIAN_POINT('Ctrl Pts',(3.48709784545464,-0.807022253075337,
-8.21070714076598));
#30973=CARTESIAN_POINT('Ctrl Pts',(3.17397693518095,-1.81503765597115,-8.12680664572484));
#30974=CARTESIAN_POINT('Ctrl Pts',(2.10722321781481,-2.98656127513204,-7.84097084863369));
#30975=CARTESIAN_POINT('Ctrl Pts',(0.644093737077059,-3.59794703410771,
-7.44892648584784));
#30976=CARTESIAN_POINT('Ctrl Pts',(-0.940587624755193,-3.53150361961666,
-7.02431239468424));
#30977=CARTESIAN_POINT('Ctrl Pts',(-2.34824590904148,-2.80195756346098,
-6.64713149419075));
#30978=CARTESIAN_POINT('Ctrl Pts',(-3.31337568314359,-1.54542548618259,
-6.38852575062885));
#30979=CARTESIAN_POINT('Ctrl Pts',(-3.54204445042266,-0.515273006800461,
-6.32725413910221));
#30980=CARTESIAN_POINT('Ctrl Pts',(-3.54204445042266,1.13787009487452E-15,
-6.32725413910221));
#30981=CARTESIAN_POINT('',(-3.54204445042266,4.33265761729611E-16,-6.32725413910221));
#30982=CARTESIAN_POINT('Ctrl Pts',(3.52930197713685,-0.299999992182585,
-8.22201570376749));
#30983=CARTESIAN_POINT('Ctrl Pts',(3.48577865853309,-0.811262373829621,
-8.21035366569568));
#30984=CARTESIAN_POINT('Ctrl Pts',(3.17248084817531,-1.81668067931843,-8.12640577041987));
#30985=CARTESIAN_POINT('Ctrl Pts',(2.10722321781481,-2.98656127513204,-7.84097084863369));
#30986=CARTESIAN_POINT('Ctrl Pts',(0.644093737077059,-3.59794703410771,
-7.44892648584784));
#30987=CARTESIAN_POINT('Ctrl Pts',(-0.940587624755193,-3.53150361961666,
-7.02431239468424));
#30988=CARTESIAN_POINT('Ctrl Pts',(-2.34824590904148,-2.80195756346098,
-6.64713149419075));
#30989=CARTESIAN_POINT('Ctrl Pts',(-3.31337568314359,-1.54542548618259,
-6.38852575062885));
#30990=CARTESIAN_POINT('Ctrl Pts',(-3.54204445042266,-0.515273006800461,
-6.32725413910221));
#30991=CARTESIAN_POINT('Ctrl Pts',(-3.54204445042266,1.13787009487452E-15,
-6.32725413910221));
#30992=CARTESIAN_POINT('',(-3.6,-4.40872847693047E-16,-6.37172499639606));
#30993=CARTESIAN_POINT('',(-3.6,1.15784830776718E-15,-6.37172499639606));
#30994=CARTESIAN_POINT('Ctrl Pts',(-3.6,1.15784830776718E-15,-6.37172499639606));
#30995=CARTESIAN_POINT('Ctrl Pts',(-3.6,-0.521978420795187,-6.37172499639606));
#30996=CARTESIAN_POINT('Ctrl Pts',(-3.36945925169178,-1.56555438904003,
-6.43378922985514));
#30997=CARTESIAN_POINT('Ctrl Pts',(-2.39520557608279,-2.84138111621991,
-6.69582652891509));
#30998=CARTESIAN_POINT('Ctrl Pts',(-0.970794977809144,-3.58699051730416,
-7.0783176016057));
#30999=CARTESIAN_POINT('Ctrl Pts',(0.638165371196739,-3.66186103320656,
-7.50952634922024));
#31000=CARTESIAN_POINT('Ctrl Pts',(2.12984786621321,-3.04615572678008,-7.90851029361343));
#31001=CARTESIAN_POINT('Ctrl Pts',(3.22201167914007,-1.85462953693043,-8.20013753826912));
#31002=CARTESIAN_POINT('Ctrl Pts',(3.54359058486425,-0.824819819394348,
-8.28591130419311));
#31003=CARTESIAN_POINT('Ctrl Pts',(3.58747822293043,-0.299999999999847,
-8.29761887140429));
#31004=CARTESIAN_POINT('Origin',(0.,0.,-9.175));
#31005=CARTESIAN_POINT('',(1.8,2.20436423846524E-16,-9.15));
#31006=CARTESIAN_POINT('',(1.825,-2.23498040844392E-16,-9.175));
#31007=CARTESIAN_POINT('',(-1.8,-2.20436423846524E-16,-9.15));
#31008=CARTESIAN_POINT('Origin',(0.,0.,-9.15));
#31009=CARTESIAN_POINT('Origin',(0.,0.,-9.15));
#31010=CARTESIAN_POINT('Origin',(0.,0.,-7.1));
#31011=CARTESIAN_POINT('',(-1.8,5.78924153883589E-16,-6.85403354277208));
#31012=CARTESIAN_POINT('Ctrl Pts',(-1.8,5.78924153883589E-16,-6.85403354277208));
#31013=CARTESIAN_POINT('Ctrl Pts',(-1.8,0.26687426398062,-6.85403354277208));
#31014=CARTESIAN_POINT('Ctrl Pts',(-1.67940772680176,0.799740126243808,
-6.88664705235894));
#31015=CARTESIAN_POINT('Ctrl Pts',(-1.11413450545355,1.51982118043229,-7.03926580415177));
#31016=CARTESIAN_POINT('Ctrl Pts',(-0.334475738167088,1.83326108962433,
-7.24892365218508));
#31017=CARTESIAN_POINT('Ctrl Pts',(0.573750176357548,1.77351582314255,-7.49212349822523));
#31018=CARTESIAN_POINT('Ctrl Pts',(1.22793100737407,1.40256541091616,-7.66657535429114));
#31019=CARTESIAN_POINT('Ctrl Pts',(1.74830857687837,0.648316915010969,-7.80494537493236));
#31020=CARTESIAN_POINT('Ctrl Pts',(1.86228369146514,-0.0991722029991063,
-7.83518501898388));
#31021=CARTESIAN_POINT('Ctrl Pts',(1.58921257783203,-0.975508826078887,
-7.76267099529992));
#31022=CARTESIAN_POINT('Ctrl Pts',(1.0724332556989,-1.52476364806832,-7.62518482796827));
#31023=CARTESIAN_POINT('Ctrl Pts',(0.305930130124348,-1.81739157595408,
-7.42046869575053));
#31024=CARTESIAN_POINT('Ctrl Pts',(-0.429751697338143,-1.81110956273029,
-7.22333465973037));
#31025=CARTESIAN_POINT('Ctrl Pts',(-1.17066142134837,-1.44648931941929,
-7.02399504594777));
#31026=CARTESIAN_POINT('Ctrl Pts',(-1.6794416245078,-0.800547883395893,
-6.88664347771834));
#31027=CARTESIAN_POINT('Ctrl Pts',(-1.8,-0.26687426398062,-6.85403354277208));
#31028=CARTESIAN_POINT('Ctrl Pts',(-1.8,-2.20436423846524E-16,-6.85403354277208));
#31029=CARTESIAN_POINT('',(-1.8,-2.20436423846524E-16,-7.1));
#31030=CARTESIAN_POINT('Ctrl Pts',(-3.6,1.15784830776718E-15,-6.37172499639606));
#31031=CARTESIAN_POINT('Ctrl Pts',(-3.6,0.521978420795508,-6.37172499639606));
#31032=CARTESIAN_POINT('Ctrl Pts',(-3.3694145818453,1.56557914338224,-6.4338013249984));
#31033=CARTESIAN_POINT('Ctrl Pts',(-2.39509191806484,2.84110705316819,-6.69585623025017));
#31034=CARTESIAN_POINT('Ctrl Pts',(-0.970891104391535,3.58753956045663,
-7.07829389448567));
#31035=CARTESIAN_POINT('Ctrl Pts',(0.638073973195017,3.66128730235917,-7.50949972707459));
#31036=CARTESIAN_POINT('Ctrl Pts',(2.13014841105312,3.04667385631827,-7.90859191608972));
#31037=CARTESIAN_POINT('Ctrl Pts',(3.22176591600978,1.85431823154204,-8.20007153069477));
#31038=CARTESIAN_POINT('Ctrl Pts',(3.54359058486578,0.824819819388012,-8.28591130419351));
#31039=CARTESIAN_POINT('Ctrl Pts',(3.587478222931,0.299999999993108,-8.29761887140444));
#31040=CARTESIAN_POINT('Ctrl Pts',(-3.58068148347422,9.16320792421322E-16,
-6.35690137729811));
#31041=CARTESIAN_POINT('Ctrl Pts',(-3.58068148347422,0.519743282797265,
-6.35690137729811));
#31042=CARTESIAN_POINT('Ctrl Pts',(-3.3507196921498,1.55886868196113,-6.4187135549211));
#31043=CARTESIAN_POINT('Ctrl Pts',(-2.37944049713545,2.82796548033986,-6.67962432039998));
#31044=CARTESIAN_POINT('Ctrl Pts',(-0.960817466988908,3.56904327507393,
-7.06029268659327));
#31045=CARTESIAN_POINT('Ctrl Pts',(0.640044730645557,3.63998643185216,-7.48929904590942));
#31046=CARTESIAN_POINT('Ctrl Pts',(2.1226102634193,3.0267995387376,-7.88607931537165));
#31047=CARTESIAN_POINT('Ctrl Pts',(3.20575390993616,1.8411284699177,-8.17562783788156));
#31048=CARTESIAN_POINT('Ctrl Pts',(3.52475967172923,0.81888729728172,-8.2608432497178));
#31049=CARTESIAN_POINT('Ctrl Pts',(3.56826802079117,0.297839652197537,-8.27246655006872));
#31050=CARTESIAN_POINT('Ctrl Pts',(-3.56136296694844,6.74793277075467E-16,
-6.34207775820016));
#31051=CARTESIAN_POINT('Ctrl Pts',(-3.56136296694844,0.517508144799021,
-6.34207775820016));
#31052=CARTESIAN_POINT('Ctrl Pts',(-3.33202480245431,1.55215822054003,-6.4036257848438));
#31053=CARTESIAN_POINT('Ctrl Pts',(-2.36378907620607,2.81482390751152,-6.66339241054979));
#31054=CARTESIAN_POINT('Ctrl Pts',(-0.950743829586281,3.55054698969123,
-7.04229147870087));
#31055=CARTESIAN_POINT('Ctrl Pts',(0.642015488096099,3.61868556134514,-7.46909836474424));
#31056=CARTESIAN_POINT('Ctrl Pts',(2.11507211578549,3.00692522115694,-7.86356671465357));
#31057=CARTESIAN_POINT('Ctrl Pts',(3.18974190386254,1.82793870829337,-8.15118414506835));
#31058=CARTESIAN_POINT('Ctrl Pts',(3.50592875859267,0.812954775175428,-8.23577519524209));
#31059=CARTESIAN_POINT('Ctrl Pts',(3.54905781865134,0.295679304401967,-8.247314228733));
#31060=CARTESIAN_POINT('Ctrl Pts',(-3.54204445042266,4.33265761729611E-16,
-6.32725413910221));
#31061=CARTESIAN_POINT('Ctrl Pts',(-3.54204445042266,0.515273006800777,
-6.32725413910221));
#31062=CARTESIAN_POINT('Ctrl Pts',(-3.31332991275881,1.54544775911892,-6.3885380147665));
#31063=CARTESIAN_POINT('Ctrl Pts',(-2.34813765527668,2.80168233468319,-6.6471605006996));
#31064=CARTESIAN_POINT('Ctrl Pts',(-0.940670192183654,3.53205070430853,
-7.02429027080846));
#31065=CARTESIAN_POINT('Ctrl Pts',(0.643986245546639,3.59738469083813,-7.44889768357907));
#31066=CARTESIAN_POINT('Ctrl Pts',(2.10753396815167,2.98705090357626,-7.8410541139355));
#31067=CARTESIAN_POINT('Ctrl Pts',(3.17372989778892,1.81474894666904,-8.12674045225515));
#31068=CARTESIAN_POINT('Ctrl Pts',(3.48709784545612,0.807022253069137,-8.21070714076638));
#31069=CARTESIAN_POINT('Ctrl Pts',(3.52984761651152,0.293518956606396,-8.22216190739728));
#31070=CARTESIAN_POINT('Ctrl Pts',(3.587478222931,0.299999999993108,-8.29761887140444));
#31071=CARTESIAN_POINT('Ctrl Pts',(3.54359058486578,0.824819819388012,-8.28591130419351));
#31072=CARTESIAN_POINT('Ctrl Pts',(3.22176591600978,1.85431823154204,-8.20007153069477));
#31073=CARTESIAN_POINT('Ctrl Pts',(2.13014841105312,3.04667385631827,-7.90859191608972));
#31074=CARTESIAN_POINT('Ctrl Pts',(0.638073973195017,3.66128730235917,-7.50949972707459));
#31075=CARTESIAN_POINT('Ctrl Pts',(-0.970891104391535,3.58753956045663,
-7.07829389448567));
#31076=CARTESIAN_POINT('Ctrl Pts',(-2.39509191806484,2.84110705316819,-6.69585623025017));
#31077=CARTESIAN_POINT('Ctrl Pts',(-3.3694145818453,1.56557914338224,-6.4338013249984));
#31078=CARTESIAN_POINT('Ctrl Pts',(-3.6,0.521978420795508,-6.37172499639606));
#31079=CARTESIAN_POINT('Ctrl Pts',(-3.6,1.15784830776718E-15,-6.37172499639606));
#31080=CARTESIAN_POINT('Ctrl Pts',(-3.54204445042266,4.33265761729611E-16,
-6.32725413910221));
#31081=CARTESIAN_POINT('Ctrl Pts',(-3.54204445042266,0.515273006800777,
-6.32725413910221));
#31082=CARTESIAN_POINT('Ctrl Pts',(-3.31332991275881,1.54544775911892,-6.3885380147665));
#31083=CARTESIAN_POINT('Ctrl Pts',(-2.34813765527668,2.80168233468319,-6.6471605006996));
#31084=CARTESIAN_POINT('Ctrl Pts',(-0.940670192183654,3.53205070430853,
-7.02429027080846));
#31085=CARTESIAN_POINT('Ctrl Pts',(0.643986245546639,3.59738469083813,-7.44889768357907));
#31086=CARTESIAN_POINT('Ctrl Pts',(2.10753396815167,2.98705090357626,-7.8410541139355));
#31087=CARTESIAN_POINT('Ctrl Pts',(3.1722345914494,1.81639306338274,-8.12633978612904));
#31088=CARTESIAN_POINT('Ctrl Pts',(3.48577762046219,0.811261167252587,-8.21035338754543));
#31089=CARTESIAN_POINT('Ctrl Pts',(3.52930197000342,0.299999991525393,-8.22201570185609));
#31090=CARTESIAN_POINT('Origin',(5.,0.,-8.61608805130371));
#31091=CARTESIAN_POINT('',(-1.85795554957734,-2.2804350980996E-16,-6.77850440006593));
#31092=CARTESIAN_POINT('Ctrl Pts',(-1.85795554957734,-2.2804350980996E-16,
-6.77850440006593));
#31093=CARTESIAN_POINT('Ctrl Pts',(-1.85795554957734,-0.278571987572876,
-6.77850440006593));
#31094=CARTESIAN_POINT('Ctrl Pts',(-1.73080482781577,-0.835578184689179,
-6.81257433327898));
#31095=CARTESIAN_POINT('Ctrl Pts',(-1.19721215014567,-1.50451692895392,
-6.95555006034784));
#31096=CARTESIAN_POINT('Ctrl Pts',(-0.426813297908517,-1.87546640869451,
-7.16197781065465));
#31097=CARTESIAN_POINT('Ctrl Pts',(0.331666591879056,-1.87496444295698,
-7.36521188459848));
#31098=CARTESIAN_POINT('Ctrl Pts',(1.11729788835015,-1.56749433429653,-7.57572115603652));
#31099=CARTESIAN_POINT('Ctrl Pts',(1.64373118835486,-1.00063243714026,-7.71677853364164));
#31100=CARTESIAN_POINT('Ctrl Pts',(1.9212206160491,-0.101532313150842,-7.79113160170048));
#31101=CARTESIAN_POINT('Ctrl Pts',(1.80554343537535,0.664494087294352,-7.76013599455624));
#31102=CARTESIAN_POINT('Ctrl Pts',(1.27579391161014,1.44087268677251,-7.61819003747258));
#31103=CARTESIAN_POINT('Ctrl Pts',(0.607000118700147,1.82734856002952,-7.4389872807594));
#31104=CARTESIAN_POINT('Ctrl Pts',(-0.328153427773111,1.89732786062517,
-7.18841364318279));
#31105=CARTESIAN_POINT('Ctrl Pts',(-1.13784193049475,1.5804395186218,-6.97145826275776));
#31106=CARTESIAN_POINT('Ctrl Pts',(-1.73081608572944,0.834748528063086,
-6.8125713167301));
#31107=CARTESIAN_POINT('Ctrl Pts',(-1.85795554957734,0.278571987572876,
-6.77850440006593));
#31108=CARTESIAN_POINT('Ctrl Pts',(-1.85795554957734,2.2804350980996E-16,
-6.77850440006593));
#31109=CARTESIAN_POINT('Origin',(0.,0.,-6.8));
#31110=CARTESIAN_POINT('Origin',(0.,0.,-8.6));
#31111=CARTESIAN_POINT('Ctrl Pts',(-1.8,-2.20436423846524E-16,-6.85403354277208));
#31112=CARTESIAN_POINT('Ctrl Pts',(-1.8,-0.26687426398062,-6.85403354277208));
#31113=CARTESIAN_POINT('Ctrl Pts',(-1.6794416245078,-0.800547883395893,
-6.88664347771834));
#31114=CARTESIAN_POINT('Ctrl Pts',(-1.17066142134837,-1.44648931941929,
-7.02399504594777));
#31115=CARTESIAN_POINT('Ctrl Pts',(-0.429751697338143,-1.81110956273029,
-7.22333465973037));
#31116=CARTESIAN_POINT('Ctrl Pts',(0.305930130124348,-1.81739157595408,
-7.42046869575053));
#31117=CARTESIAN_POINT('Ctrl Pts',(1.0724332556989,-1.52476364806832,-7.62518482796827));
#31118=CARTESIAN_POINT('Ctrl Pts',(1.58921257783203,-0.975508826078887,
-7.76267099529992));
#31119=CARTESIAN_POINT('Ctrl Pts',(1.86228369146514,-0.0991722029991063,
-7.83518501898388));
#31120=CARTESIAN_POINT('Ctrl Pts',(1.74830857687837,0.648316915010969,-7.80494537493236));
#31121=CARTESIAN_POINT('Ctrl Pts',(1.22793100737407,1.40256541091616,-7.66657535429114));
#31122=CARTESIAN_POINT('Ctrl Pts',(0.573750176357548,1.77351582314255,-7.49212349822523));
#31123=CARTESIAN_POINT('Ctrl Pts',(-0.334475738167088,1.83326108962433,
-7.24892365218508));
#31124=CARTESIAN_POINT('Ctrl Pts',(-1.11413450545355,1.51982118043229,-7.03926580415177));
#31125=CARTESIAN_POINT('Ctrl Pts',(-1.67940772680176,0.799740126243808,
-6.88664705235894));
#31126=CARTESIAN_POINT('Ctrl Pts',(-1.8,0.26687426398062,-6.85403354277208));
#31127=CARTESIAN_POINT('Ctrl Pts',(-1.8,5.78924153883589E-16,-6.85403354277208));
#31128=CARTESIAN_POINT('Ctrl Pts',(-1.81931851652578,-2.22972119167669E-16,
-6.82885716187003));
#31129=CARTESIAN_POINT('Ctrl Pts',(-1.81931851652578,-0.270773505178038,
-6.82885716187003));
#31130=CARTESIAN_POINT('Ctrl Pts',(-1.69656269227712,-0.812224650493655,
-6.86195376290522));
#31131=CARTESIAN_POINT('Ctrl Pts',(-1.17951166428081,-1.46583185593083,
-7.00118005074779));
#31132=CARTESIAN_POINT('Ctrl Pts',(-0.428772230861601,-1.83256184471836,
-7.20288237670513));
#31133=CARTESIAN_POINT('Ctrl Pts',(0.314508950709251,-1.83658253162171,
-7.40204975869984));
#31134=CARTESIAN_POINT('Ctrl Pts',(1.08738813324932,-1.53900721014439,-7.60869693732435));
#31135=CARTESIAN_POINT('Ctrl Pts',(1.60738544800631,-0.983883363099342,
-7.74737350808049));
#31136=CARTESIAN_POINT('Ctrl Pts',(1.88192933299313,-0.0999589063830184,
-7.82050054655608));
#31137=CARTESIAN_POINT('Ctrl Pts',(1.76738686304403,0.653709305772098,-7.79000891480699));
#31138=CARTESIAN_POINT('Ctrl Pts',(1.24388530878609,1.41533450286828,-7.65044691535163));
#31139=CARTESIAN_POINT('Ctrl Pts',(0.584833490471748,1.79146006877154,-7.47441142573662));
#31140=CARTESIAN_POINT('Ctrl Pts',(-0.332368301369096,1.85461667995794,
-7.22875364918432));
#31141=CARTESIAN_POINT('Ctrl Pts',(-1.12203698046728,1.54002729316212,-7.01666329035377));
#31142=CARTESIAN_POINT('Ctrl Pts',(-1.69654384644432,0.811409593516901,
-6.86195514048266));
#31143=CARTESIAN_POINT('Ctrl Pts',(-1.81931851652578,0.270773505178039,
-6.82885716187003));
#31144=CARTESIAN_POINT('Ctrl Pts',(-1.81931851652578,4.61963939192379E-16,
-6.82885716187003));
#31145=CARTESIAN_POINT('Ctrl Pts',(-1.83863703305156,-2.25507814488814E-16,
-6.80368078096798));
#31146=CARTESIAN_POINT('Ctrl Pts',(-1.83863703305156,-0.274672746375458,
-6.80368078096798));
#31147=CARTESIAN_POINT('Ctrl Pts',(-1.71368376004645,-0.823901417591417,
-6.83726404809209));
#31148=CARTESIAN_POINT('Ctrl Pts',(-1.18836190721324,-1.48517439244238,
-6.97836505554782));
#31149=CARTESIAN_POINT('Ctrl Pts',(-0.427792764385059,-1.85401412670644,
-7.18243009367989));
#31150=CARTESIAN_POINT('Ctrl Pts',(0.323087771294154,-1.85577348728935,
-7.38363082164916));
#31151=CARTESIAN_POINT('Ctrl Pts',(1.10234301079973,-1.55325077222046,-7.59220904668044));
#31152=CARTESIAN_POINT('Ctrl Pts',(1.62555831818059,-0.9922579001198,-7.73207602086106));
#31153=CARTESIAN_POINT('Ctrl Pts',(1.90157497452111,-0.10074560976693,-7.80581607412828));
#31154=CARTESIAN_POINT('Ctrl Pts',(1.78646514920969,0.659101696533225,-7.77507245468161));
#31155=CARTESIAN_POINT('Ctrl Pts',(1.25983961019812,1.42810359482039,-7.6343184764121));
#31156=CARTESIAN_POINT('Ctrl Pts',(0.595916804585947,1.80940431440053,-7.45669935324801));
#31157=CARTESIAN_POINT('Ctrl Pts',(-0.330260864571104,1.87597227029155,
-7.20858364618355));
#31158=CARTESIAN_POINT('Ctrl Pts',(-1.12993945548101,1.56023340589196,-6.99406077655577));
#31159=CARTESIAN_POINT('Ctrl Pts',(-1.71367996608688,0.823079060789994,
-6.83726322860638));
#31160=CARTESIAN_POINT('Ctrl Pts',(-1.83863703305156,0.274672746375458,
-6.80368078096798));
#31161=CARTESIAN_POINT('Ctrl Pts',(-1.83863703305156,3.4500372450117E-16,
-6.80368078096798));
#31162=CARTESIAN_POINT('Ctrl Pts',(-1.85795554957734,-2.2804350980996E-16,
-6.77850440006593));
#31163=CARTESIAN_POINT('Ctrl Pts',(-1.85795554957734,-0.278571987572876,
-6.77850440006593));
#31164=CARTESIAN_POINT('Ctrl Pts',(-1.73080482781577,-0.835578184689179,
-6.81257433327898));
#31165=CARTESIAN_POINT('Ctrl Pts',(-1.19721215014567,-1.50451692895392,
-6.95555006034784));
#31166=CARTESIAN_POINT('Ctrl Pts',(-0.426813297908517,-1.87546640869451,
-7.16197781065465));
#31167=CARTESIAN_POINT('Ctrl Pts',(0.331666591879056,-1.87496444295698,
-7.36521188459848));
#31168=CARTESIAN_POINT('Ctrl Pts',(1.11729788835015,-1.56749433429653,-7.57572115603652));
#31169=CARTESIAN_POINT('Ctrl Pts',(1.64373118835486,-1.00063243714026,-7.71677853364164));
#31170=CARTESIAN_POINT('Ctrl Pts',(1.9212206160491,-0.101532313150842,-7.79113160170048));
#31171=CARTESIAN_POINT('Ctrl Pts',(1.80554343537535,0.664494087294352,-7.76013599455624));
#31172=CARTESIAN_POINT('Ctrl Pts',(1.27579391161014,1.44087268677251,-7.61819003747258));
#31173=CARTESIAN_POINT('Ctrl Pts',(0.607000118700147,1.82734856002952,-7.4389872807594));
#31174=CARTESIAN_POINT('Ctrl Pts',(-0.328153427773111,1.89732786062517,
-7.18841364318279));
#31175=CARTESIAN_POINT('Ctrl Pts',(-1.13784193049475,1.5804395186218,-6.97145826275776));
#31176=CARTESIAN_POINT('Ctrl Pts',(-1.73081608572944,0.834748528063086,
-6.8125713167301));
#31177=CARTESIAN_POINT('Ctrl Pts',(-1.85795554957734,0.278571987572876,
-6.77850440006593));
#31178=CARTESIAN_POINT('Ctrl Pts',(-1.85795554957734,2.2804350980996E-16,
-6.77850440006593));
#31179=CARTESIAN_POINT('',(-1.8,-2.20436423846524E-16,-6.85403354277208));
#31180=CARTESIAN_POINT('Origin',(0.,0.,-8.89));
#31181=CARTESIAN_POINT('Origin',(0.,0.,-8.66));
#31182=CARTESIAN_POINT('Origin',(0.,0.,-8.63));
#31183=CARTESIAN_POINT('Origin',(0.,0.,-8.6));
#31184=CARTESIAN_POINT('Origin',(3.6,0.,-8.6));
#59164=UNCERTAINTY_MEASURE_WITH_UNIT(LENGTH_MEASURE(0.001),#59205,
'DISTANCE_ACCURACY_VALUE',
'Maximum model space distance between geometric entities at asserted c
onnectivities');
#59182=UNCERTAINTY_MEASURE_WITH_UNIT(LENGTH_MEASURE(0.001),#59205,
'DISTANCE_ACCURACY_VALUE',
'Maximum model space distance between geometric entities at asserted c
onnectivities');
#59186=(
GEOMETRIC_REPRESENTATION_CONTEXT(3)
GLOBAL_UNCERTAINTY_ASSIGNED_CONTEXT((#59164))
GLOBAL_UNIT_ASSIGNED_CONTEXT((#59205,#59207,#59208))
REPRESENTATION_CONTEXT('','3D')
);
#59204=(
GEOMETRIC_REPRESENTATION_CONTEXT(3)
GLOBAL_UNCERTAINTY_ASSIGNED_CONTEXT((#59182))
GLOBAL_UNIT_ASSIGNED_CONTEXT((#59205,#59207,#59208))
REPRESENTATION_CONTEXT('','3D')
);
#59205=(
LENGTH_UNIT()
NAMED_UNIT(*)
SI_UNIT(.CENTI.,.METRE.)
);
#59207=(
NAMED_UNIT(*)
PLANE_ANGLE_UNIT()
SI_UNIT($,.RADIAN.)
);
#59208=(
NAMED_UNIT(*)
SI_UNIT($,.STERADIAN.)
SOLID_ANGLE_UNIT()
);
#59212=SHAPE_DEFINITION_REPRESENTATION(#59233,#59299);
#59233=PRODUCT_DEFINITION_SHAPE('',$,#59321);
#59299=SHAPE_REPRESENTATION('',(#23145),#59186);
#59317=PRODUCT_DEFINITION_CONTEXT('part definition',#59382,'design');
#59321=PRODUCT_DEFINITION('2026-10-23-00-47-19-372',
'10_Swashplate_15deg',#59342,#59317);
#59342=PRODUCT_DEFINITION_FORMATION('',$,#59387);
#59382=APPLICATION_CONTEXT(
'Core Data for Automotive Mechanical Design Process');
#59383=PRODUCT_CONTEXT('part definition',#59382,'mechanical');
#59387=PRODUCT('2026-10-23-00-47-19-372','10_Swashplate_15deg',$,(#59383));
#59566=COLOUR_RGB('Light Blue',0.38,0.62,0.78);
#59567=FILL_AREA_STYLE_COLOUR('',#59566);
#59568=FILL_AREA_STYLE('',(#59567));
#59569=SURFACE_STYLE_FILL_AREA(#59568);
#59570=SURFACE_SIDE_STYLE('',(#59569));
#59571=SURFACE_STYLE_USAGE(.BOTH.,#59570);
#59572=PRESENTATION_STYLE_ASSIGNMENT((#59571));
ENDSEC;
END-ISO-10303-21;
